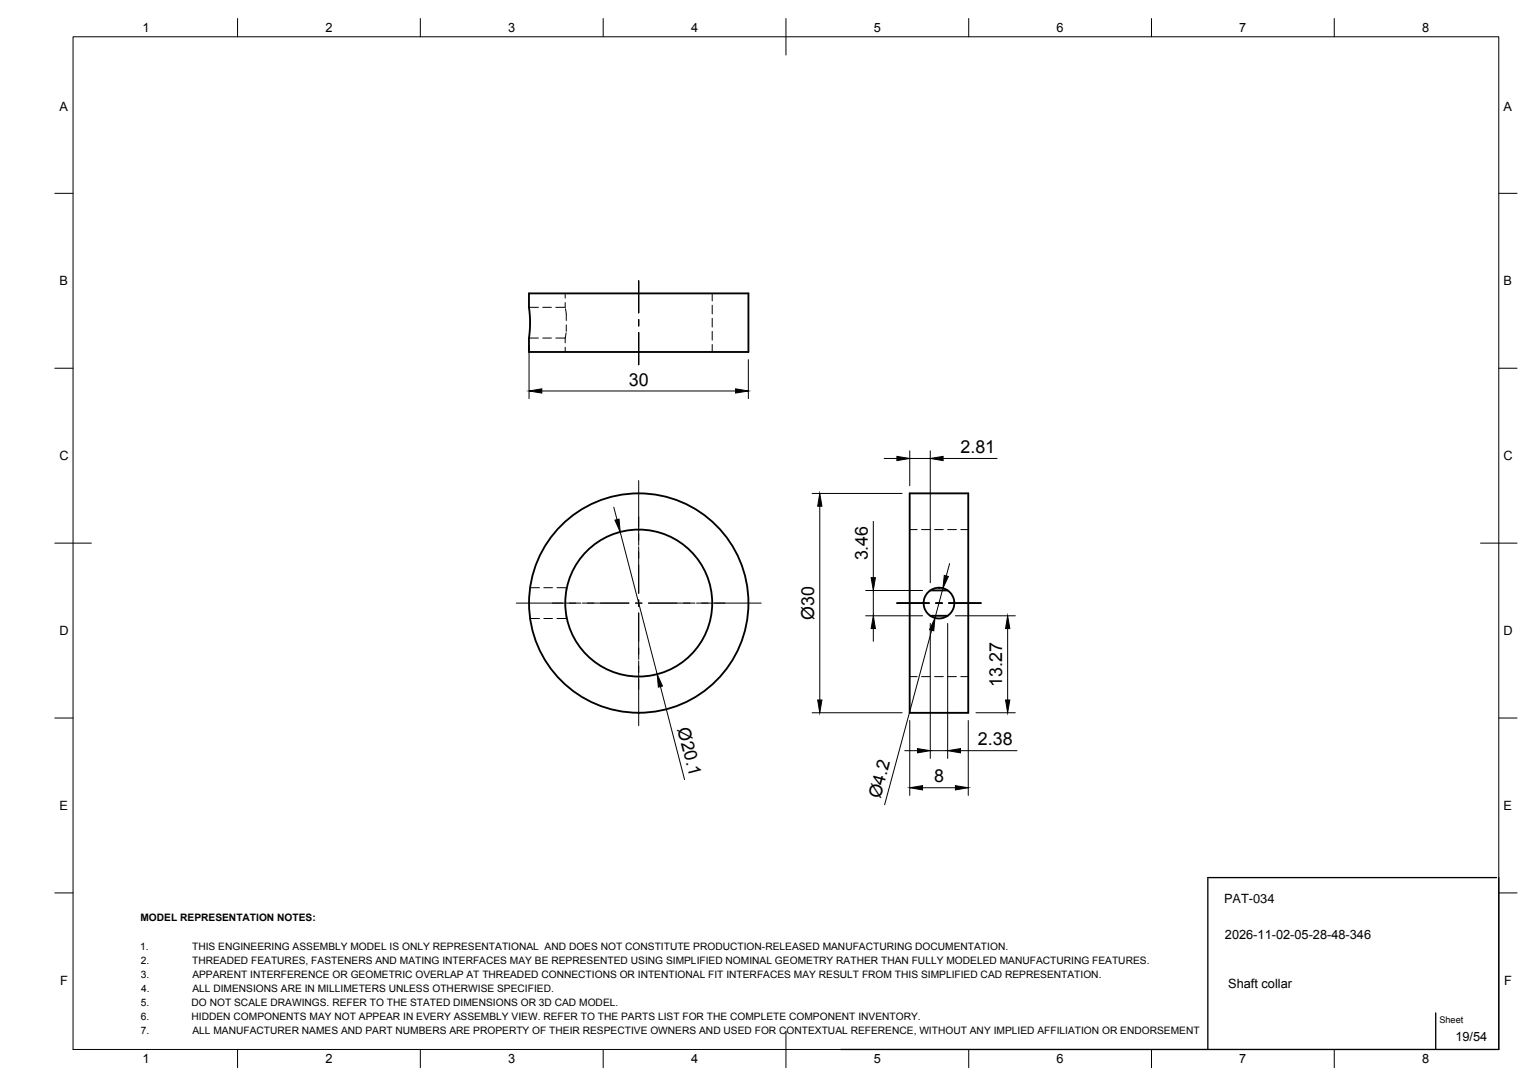
ISO-10303-21;
HEADER;
/* Generated by software containing ST-Developer
 * from STEP Tools, Inc. (www.steptools.com) 
 */

FILE_DESCRIPTION(
/* description */ ('Fatigue rig crank-slider'),
/* implementation_level */ '2;1');

FILE_NAME(
/* name */ 'Shaft collar.step',
/* time_stamp */ '2026-10-28T03:24:50-07:00',
/* author */ (''),
/* organization */ (''),
/* preprocessor_version */ 'ST-DEVELOPER v20.2',
/* originating_system */ 'Autodesk Translation Framework v15.17.0.0',
/* authorisation */ '');

FILE_SCHEMA (('AUTOMOTIVE_DESIGN { 1 0 10303 214 3 1 1 }'));
ENDSEC;

DATA;
#10=MECHANICAL_DESIGN_GEOMETRIC_PRESENTATION_REPRESENTATION('',(#605),#16911);
#439=B_SPLINE_CURVE_WITH_KNOTS('',3,(#14824,#14825,#14826,#14827,#14828,
#14829,#14830,#14831,#14832,#14833,#14834,#14835,#14836,#14837),
 .UNSPECIFIED.,.F.,.F.,(4,2,2,2,2,2,4),(0.756005737987026,0.793568827564645,
0.8729225200542,0.952276212543755,1.03162990503331,1.11098359752287,1.14854668710048),
 .UNSPECIFIED.);
#440=B_SPLINE_CURVE_WITH_KNOTS('',3,(#14843,#14844,#14845,#14846,#14847,
#14848,#14849,#14850,#14851,#14852,#14853,#14854,#14855,#14856,#14857,#14858,
#14859,#14860),.UNSPECIFIED.,.F.,.F.,(4,2,2,2,2,2,2,2,4),(0.,0.0792165807733624,
0.158433161546725,0.23764869707457,0.316864232602414,0.396079768130259,
0.475295303658103,0.554511884431466,0.633728465204828),.UNSPECIFIED.);
#441=B_SPLINE_CURVE_WITH_KNOTS('',3,(#14861,#14862,#14863,#14864,#14865,
#14866,#14867,#14868,#14869,#14870,#14871,#14872,#14873,#14874,#14875,#14876,
#14877,#14878),.UNSPECIFIED.,.F.,.F.,(4,2,2,2,2,2,2,2,4),(0.633728465204828,
0.712945045978191,0.792161626751553,0.871377162279398,0.950592697807242,
1.02980823333509,1.10902376886293,1.18824034963629,1.26745693040966),
 .UNSPECIFIED.);
#442=B_SPLINE_CURVE_WITH_KNOTS('',3,(#14881,#14882,#14883,#14884,#14885,
#14886,#14887,#14888,#14889,#14890,#14891,#14892,#14893,#14894),
 .UNSPECIFIED.,.F.,.F.,(4,2,2,2,2,2,4),(0.121154929624525,0.158718019202141,
0.238071711691697,0.317425404181252,0.396779096670807,0.476132789160362,
0.513695878737981),.UNSPECIFIED.);
#504=SHAPE_REPRESENTATION_RELATIONSHIP('SRR','None',#17145,#554);
#554=ADVANCED_BREP_SHAPE_REPRESENTATION('',(#662),#16874);
#605=STYLED_ITEM('',(#17487),#662);
#662=MANIFOLD_SOLID_BREP('Body1',#8898);
#821=FACE_BOUND('',#2092,.T.);
#822=FACE_BOUND('',#2094,.T.);
#823=FACE_BOUND('',#2096,.T.);
#824=FACE_BOUND('',#2098,.T.);
#1033=PLANE('',#9913);
#1034=PLANE('',#9918);
#1035=PLANE('',#9925);
#1036=PLANE('',#9926);
#1444=FACE_OUTER_BOUND('',#2088,.T.);
#1445=FACE_OUTER_BOUND('',#2089,.T.);
#1446=FACE_OUTER_BOUND('',#2090,.T.);
#1447=FACE_OUTER_BOUND('',#2091,.T.);
#1448=FACE_OUTER_BOUND('',#2093,.T.);
#1449=FACE_OUTER_BOUND('',#2095,.T.);
#1450=FACE_OUTER_BOUND('',#2097,.T.);
#2088=EDGE_LOOP('',(#6950,#6951));
#2089=EDGE_LOOP('',(#6952,#6953,#6954,#6955,#6956,#6957,#6958,#6959,#6960));
#2090=EDGE_LOOP('',(#6961,#6962,#6963));
#2091=EDGE_LOOP('',(#6964,#6965,#6966,#6967));
#2092=EDGE_LOOP('',(#6968,#6969,#6970,#6971));
#2093=EDGE_LOOP('',(#6972,#6973,#6974,#6975));
#2094=EDGE_LOOP('',(#6976,#6977));
#2095=EDGE_LOOP('',(#6978));
#2096=EDGE_LOOP('',(#6979));
#2097=EDGE_LOOP('',(#6980));
#2098=EDGE_LOOP('',(#6981));
#2744=LINE('',#14820,#3390);
#2745=LINE('',#14841,#3391);
#2746=LINE('',#14896,#3392);
#2747=LINE('',#14901,#3393);
#2748=LINE('',#14907,#3394);
#3390=VECTOR('',#11692,1.);
#3391=VECTOR('',#11699,0.21);
#3392=VECTOR('',#11704,1.);
#3393=VECTOR('',#11709,1.005);
#3394=VECTOR('',#11716,1.5);
#3921=CIRCLE('',#9914,0.21);
#3922=CIRCLE('',#9916,0.21);
#3923=CIRCLE('',#9917,0.21);
#3924=CIRCLE('',#9920,1.005);
#3925=CIRCLE('',#9921,1.005);
#3926=CIRCLE('',#9923,1.5);
#3927=CIRCLE('',#9924,1.5);
#4475=VERTEX_POINT('',#14818);
#4476=VERTEX_POINT('',#14819);
#4477=VERTEX_POINT('',#14823);
#4478=VERTEX_POINT('',#14838);
#4479=VERTEX_POINT('',#14840);
#4480=VERTEX_POINT('',#14842);
#4481=VERTEX_POINT('',#14879);
#4482=VERTEX_POINT('',#14898);
#4483=VERTEX_POINT('',#14900);
#4484=VERTEX_POINT('',#14904);
#4485=VERTEX_POINT('',#14906);
#5373=EDGE_CURVE('',#4475,#4476,#2744,.T.);
#5374=EDGE_CURVE('',#4475,#4476,#3921,.T.);
#5375=EDGE_CURVE('',#4477,#4475,#439,.T.);
#5376=EDGE_CURVE('',#4478,#4477,#3922,.T.);
#5377=EDGE_CURVE('',#4478,#4479,#2745,.T.);
#5378=EDGE_CURVE('',#4480,#4479,#440,.T.);
#5379=EDGE_CURVE('',#4479,#4480,#441,.T.);
#5380=EDGE_CURVE('',#4481,#4478,#3923,.T.);
#5381=EDGE_CURVE('',#4476,#4481,#442,.T.);
#5382=EDGE_CURVE('',#4481,#4477,#2746,.T.);
#5383=EDGE_CURVE('',#4482,#4482,#3924,.T.);
#5384=EDGE_CURVE('',#4482,#4483,#2747,.T.);
#5385=EDGE_CURVE('',#4483,#4483,#3925,.T.);
#5386=EDGE_CURVE('',#4484,#4484,#3926,.T.);
#5387=EDGE_CURVE('',#4484,#4485,#2748,.T.);
#5388=EDGE_CURVE('',#4485,#4485,#3927,.T.);
#6950=ORIENTED_EDGE('',*,*,#5373,.F.);
#6951=ORIENTED_EDGE('',*,*,#5374,.T.);
#6952=ORIENTED_EDGE('',*,*,#5375,.F.);
#6953=ORIENTED_EDGE('',*,*,#5376,.F.);
#6954=ORIENTED_EDGE('',*,*,#5377,.T.);
#6955=ORIENTED_EDGE('',*,*,#5378,.F.);
#6956=ORIENTED_EDGE('',*,*,#5379,.F.);
#6957=ORIENTED_EDGE('',*,*,#5377,.F.);
#6958=ORIENTED_EDGE('',*,*,#5380,.F.);
#6959=ORIENTED_EDGE('',*,*,#5381,.F.);
#6960=ORIENTED_EDGE('',*,*,#5374,.F.);
#6961=ORIENTED_EDGE('',*,*,#5382,.F.);
#6962=ORIENTED_EDGE('',*,*,#5380,.T.);
#6963=ORIENTED_EDGE('',*,*,#5376,.T.);
#6964=ORIENTED_EDGE('',*,*,#5383,.F.);
#6965=ORIENTED_EDGE('',*,*,#5384,.T.);
#6966=ORIENTED_EDGE('',*,*,#5385,.T.);
#6967=ORIENTED_EDGE('',*,*,#5384,.F.);
#6968=ORIENTED_EDGE('',*,*,#5381,.T.);
#6969=ORIENTED_EDGE('',*,*,#5382,.T.);
#6970=ORIENTED_EDGE('',*,*,#5375,.T.);
#6971=ORIENTED_EDGE('',*,*,#5373,.T.);
#6972=ORIENTED_EDGE('',*,*,#5386,.F.);
#6973=ORIENTED_EDGE('',*,*,#5387,.T.);
#6974=ORIENTED_EDGE('',*,*,#5388,.T.);
#6975=ORIENTED_EDGE('',*,*,#5387,.F.);
#6976=ORIENTED_EDGE('',*,*,#5378,.T.);
#6977=ORIENTED_EDGE('',*,*,#5379,.T.);
#6978=ORIENTED_EDGE('',*,*,#5386,.T.);
#6979=ORIENTED_EDGE('',*,*,#5383,.T.);
#6980=ORIENTED_EDGE('',*,*,#5388,.F.);
#6981=ORIENTED_EDGE('',*,*,#5385,.F.);
#8278=CYLINDRICAL_SURFACE('',#9915,0.21);
#8279=CYLINDRICAL_SURFACE('',#9919,1.005);
#8280=CYLINDRICAL_SURFACE('',#9922,1.5);
#8582=ADVANCED_FACE('',(#1444),#1033,.T.);
#8583=ADVANCED_FACE('',(#1445),#8278,.F.);
#8584=ADVANCED_FACE('',(#1446),#1034,.T.);
#8585=ADVANCED_FACE('',(#1447,#821),#8279,.F.);
#8586=ADVANCED_FACE('',(#1448,#822),#8280,.T.);
#8587=ADVANCED_FACE('',(#1449,#823),#1035,.T.);
#8588=ADVANCED_FACE('',(#1450,#824),#1036,.F.);
#8898=CLOSED_SHELL('',(#8582,#8583,#8584,#8585,#8586,#8587,#8588));
#9912=AXIS2_PLACEMENT_3D('',#14816,#11688,#11689);
#9913=AXIS2_PLACEMENT_3D('',#14817,#11690,#11691);
#9914=AXIS2_PLACEMENT_3D('',#14821,#11693,#11694);
#9915=AXIS2_PLACEMENT_3D('',#14822,#11695,#11696);
#9916=AXIS2_PLACEMENT_3D('',#14839,#11697,#11698);
#9917=AXIS2_PLACEMENT_3D('',#14880,#11700,#11701);
#9918=AXIS2_PLACEMENT_3D('',#14895,#11702,#11703);
#9919=AXIS2_PLACEMENT_3D('',#14897,#11705,#11706);
#9920=AXIS2_PLACEMENT_3D('',#14899,#11707,#11708);
#9921=AXIS2_PLACEMENT_3D('',#14902,#11710,#11711);
#9922=AXIS2_PLACEMENT_3D('',#14903,#11712,#11713);
#9923=AXIS2_PLACEMENT_3D('',#14905,#11714,#11715);
#9924=AXIS2_PLACEMENT_3D('',#14908,#11717,#11718);
#9925=AXIS2_PLACEMENT_3D('',#14909,#11719,#11720);
#9926=AXIS2_PLACEMENT_3D('',#14910,#11721,#11722);
#11688=DIRECTION('axis',(0.,0.,1.));
#11689=DIRECTION('refdir',(1.,0.,0.));
#11690=DIRECTION('center_axis',(0.,0.,1.));
#11691=DIRECTION('ref_axis',(1.,0.,0.));
#11692=DIRECTION('',(0.,1.,0.));
#11693=DIRECTION('center_axis',(0.,0.,1.));
#11694=DIRECTION('ref_axis',(1.,0.,0.));
#11695=DIRECTION('center_axis',(0.,0.,1.));
#11696=DIRECTION('ref_axis',(1.,0.,0.));
#11697=DIRECTION('center_axis',(0.,0.,1.));
#11698=DIRECTION('ref_axis',(1.,0.,0.));
#11699=DIRECTION('',(0.,0.,1.));
#11700=DIRECTION('center_axis',(0.,0.,1.));
#11701=DIRECTION('ref_axis',(1.,0.,0.));
#11702=DIRECTION('center_axis',(0.,0.,1.));
#11703=DIRECTION('ref_axis',(1.,0.,0.));
#11704=DIRECTION('',(0.,-1.,0.));
#11705=DIRECTION('center_axis',(0.,1.,0.));
#11706=DIRECTION('ref_axis',(1.,0.,0.));
#11707=DIRECTION('center_axis',(0.,-1.,0.));
#11708=DIRECTION('ref_axis',(1.,0.,0.));
#11709=DIRECTION('',(0.,-1.,0.));
#11710=DIRECTION('center_axis',(0.,-1.,0.));
#11711=DIRECTION('ref_axis',(1.,0.,0.));
#11712=DIRECTION('center_axis',(0.,1.,0.));
#11713=DIRECTION('ref_axis',(1.,0.,0.));
#11714=DIRECTION('center_axis',(0.,1.,0.));
#11715=DIRECTION('ref_axis',(1.,0.,0.));
#11716=DIRECTION('',(0.,-1.,0.));
#11717=DIRECTION('center_axis',(0.,1.,0.));
#11718=DIRECTION('ref_axis',(1.,0.,0.));
#11719=DIRECTION('center_axis',(0.,1.,0.));
#11720=DIRECTION('ref_axis',(1.,0.,0.));
#11721=DIRECTION('center_axis',(0.,1.,0.));
#11722=DIRECTION('ref_axis',(1.,0.,0.));
#14816=CARTESIAN_POINT('',(0.,0.,0.));
#14817=CARTESIAN_POINT('Origin',(0.,-17.05,12.99));
#14818=CARTESIAN_POINT('',(0.172988438920051,-17.1690588089979,12.99));
#14819=CARTESIAN_POINT('',(0.172988438920051,-16.9309411910021,12.99));
#14820=CARTESIAN_POINT('',(0.172988438920051,-17.45,12.99));
#14821=CARTESIAN_POINT('Origin',(0.,-17.05,12.99));
#14822=CARTESIAN_POINT('Origin',(0.,-17.05,12.99));
#14823=CARTESIAN_POINT('',(-0.172988438920051,-17.1690588089979,12.99));
#14824=CARTESIAN_POINT('Ctrl Pts',(-0.172988438920049,-17.1690588089979,
12.99));
#14825=CARTESIAN_POINT('Ctrl Pts',(-0.165594865311309,-17.1798014223953,
12.9912919219764));
#14826=CARTESIAN_POINT('Ctrl Pts',(-0.157297138725604,-17.1896877093727,
12.992653949439));
#14827=CARTESIAN_POINT('Ctrl Pts',(-0.129892073845076,-17.2170927742533,
12.9967480843909));
#14828=CARTESIAN_POINT('Ctrl Pts',(-0.106330167759284,-17.233242056333,
12.9996958932764));
#14829=CARTESIAN_POINT('Ctrl Pts',(-0.0546129046324093,-17.2546977939649,
13.0038502947236));
#14830=CARTESIAN_POINT('Ctrl Pts',(-0.0264512308298518,-17.26,13.005));
#14831=CARTESIAN_POINT('Ctrl Pts',(0.0264512308298517,-17.26,13.005));
#14832=CARTESIAN_POINT('Ctrl Pts',(0.0546129046324092,-17.2546977939649,
13.0038502947236));
#14833=CARTESIAN_POINT('Ctrl Pts',(0.106330167759284,-17.233242056333,12.9996958932764));
#14834=CARTESIAN_POINT('Ctrl Pts',(0.129892073845076,-17.2170927742533,
12.9967480843909));
#14835=CARTESIAN_POINT('Ctrl Pts',(0.157297138725604,-17.1896877093727,
12.9926539494391));
#14836=CARTESIAN_POINT('Ctrl Pts',(0.165594865311311,-17.1798014223953,
12.9912919219764));
#14837=CARTESIAN_POINT('Ctrl Pts',(0.17298843892005,-17.1690588089979,12.99));
#14838=CARTESIAN_POINT('',(-0.21,-17.05,12.99));
#14839=CARTESIAN_POINT('Origin',(0.,-17.05,12.99));
#14840=CARTESIAN_POINT('',(-0.21,-17.05,13.4852272553384));
#14841=CARTESIAN_POINT('',(-0.21,-17.05,12.99));
#14842=CARTESIAN_POINT('',(0.21,-17.05,13.4852272553384));
#14843=CARTESIAN_POINT('Ctrl Pts',(0.21,-17.05,13.4852272553384));
#14844=CARTESIAN_POINT('Ctrl Pts',(0.21,-17.0764055269245,13.4852272553384));
#14845=CARTESIAN_POINT('Ctrl Pts',(0.204715737269596,-17.1045470740907,
13.4860041595441));
#14846=CARTESIAN_POINT('Ctrl Pts',(0.183273763036332,-17.1562762689051,
13.4888007328232));
#14847=CARTESIAN_POINT('Ctrl Pts',(0.167117923970393,-17.179866924128,13.4907789715758));
#14848=CARTESIAN_POINT('Ctrl Pts',(0.129867169887369,-17.217117678211,13.4944848114133));
#14849=CARTESIAN_POINT('Ctrl Pts',(0.106276408305765,-17.2332737100014,
13.4964545565713));
#14850=CARTESIAN_POINT('Ctrl Pts',(0.0545468514058993,-17.2547158248262,
13.4992316551565));
#14851=CARTESIAN_POINT('Ctrl Pts',(0.0264051785092816,-17.26,13.5));
#14852=CARTESIAN_POINT('Ctrl Pts',(-0.0264051785092815,-17.26,13.5));
#14853=CARTESIAN_POINT('Ctrl Pts',(-0.0545468514058992,-17.2547158248262,
13.4992316551565));
#14854=CARTESIAN_POINT('Ctrl Pts',(-0.106276408305765,-17.2332737100014,
13.4964545565713));
#14855=CARTESIAN_POINT('Ctrl Pts',(-0.129867169887368,-17.217117678211,
13.4944848114133));
#14856=CARTESIAN_POINT('Ctrl Pts',(-0.167117923970393,-17.179866924128,
13.4907789715758));
#14857=CARTESIAN_POINT('Ctrl Pts',(-0.183273763036332,-17.1562762689051,
13.4888007328232));
#14858=CARTESIAN_POINT('Ctrl Pts',(-0.204715737269596,-17.1045470740907,
13.4860041595441));
#14859=CARTESIAN_POINT('Ctrl Pts',(-0.21,-17.0764055269245,13.4852272553384));
#14860=CARTESIAN_POINT('Ctrl Pts',(-0.21,-17.05,13.4852272553384));
#14861=CARTESIAN_POINT('Ctrl Pts',(-0.21,-17.05,13.4852272553384));
#14862=CARTESIAN_POINT('Ctrl Pts',(-0.21,-17.0235944730756,13.4852272553384));
#14863=CARTESIAN_POINT('Ctrl Pts',(-0.204715737269596,-16.9954529259093,
13.4860041595441));
#14864=CARTESIAN_POINT('Ctrl Pts',(-0.183273763036332,-16.9437237310949,
13.4888007328232));
#14865=CARTESIAN_POINT('Ctrl Pts',(-0.167117923970393,-16.920133075872,
13.4907789715758));
#14866=CARTESIAN_POINT('Ctrl Pts',(-0.129867169887369,-16.882882321789,
13.4944848114133));
#14867=CARTESIAN_POINT('Ctrl Pts',(-0.106276408305765,-16.8667262899986,
13.4964545565713));
#14868=CARTESIAN_POINT('Ctrl Pts',(-0.0545468514058993,-16.8452841751738,
13.4992316551565));
#14869=CARTESIAN_POINT('Ctrl Pts',(-0.0264051785092816,-16.84,13.5));
#14870=CARTESIAN_POINT('Ctrl Pts',(0.0264051785092815,-16.84,13.5));
#14871=CARTESIAN_POINT('Ctrl Pts',(0.0545468514058992,-16.8452841751738,
13.4992316551565));
#14872=CARTESIAN_POINT('Ctrl Pts',(0.106276408305765,-16.8667262899986,
13.4964545565713));
#14873=CARTESIAN_POINT('Ctrl Pts',(0.129867169887368,-16.882882321789,13.4944848114133));
#14874=CARTESIAN_POINT('Ctrl Pts',(0.167117923970393,-16.920133075872,13.4907789715758));
#14875=CARTESIAN_POINT('Ctrl Pts',(0.183273763036332,-16.9437237310949,
13.4888007328232));
#14876=CARTESIAN_POINT('Ctrl Pts',(0.204715737269596,-16.9954529259093,
13.4860041595441));
#14877=CARTESIAN_POINT('Ctrl Pts',(0.21,-17.0235944730756,13.4852272553384));
#14878=CARTESIAN_POINT('Ctrl Pts',(0.21,-17.05,13.4852272553384));
#14879=CARTESIAN_POINT('',(-0.172988438920051,-16.9309411910021,12.99));
#14880=CARTESIAN_POINT('Origin',(0.,-17.05,12.99));
#14881=CARTESIAN_POINT('Ctrl Pts',(0.17298843892005,-16.9309411910021,12.99));
#14882=CARTESIAN_POINT('Ctrl Pts',(0.165594865311311,-16.9201985776047,
12.9912919219764));
#14883=CARTESIAN_POINT('Ctrl Pts',(0.157297138725604,-16.9103122906273,
12.992653949439));
#14884=CARTESIAN_POINT('Ctrl Pts',(0.129892073845076,-16.8829072257467,
12.9967480843909));
#14885=CARTESIAN_POINT('Ctrl Pts',(0.106330167759284,-16.8667579436671,
12.9996958932764));
#14886=CARTESIAN_POINT('Ctrl Pts',(0.0546129046324093,-16.8453022060351,
13.0038502947236));
#14887=CARTESIAN_POINT('Ctrl Pts',(0.0264512308298517,-16.84,13.005));
#14888=CARTESIAN_POINT('Ctrl Pts',(-0.0264512308298517,-16.84,13.005));
#14889=CARTESIAN_POINT('Ctrl Pts',(-0.054612904632409,-16.8453022060351,
13.0038502947236));
#14890=CARTESIAN_POINT('Ctrl Pts',(-0.106330167759284,-16.8667579436671,
12.9996958932764));
#14891=CARTESIAN_POINT('Ctrl Pts',(-0.129892073845076,-16.8829072257467,
12.9967480843909));
#14892=CARTESIAN_POINT('Ctrl Pts',(-0.157297138725604,-16.9103122906273,
12.9926539494391));
#14893=CARTESIAN_POINT('Ctrl Pts',(-0.165594865311311,-16.9201985776047,
12.9912919219764));
#14894=CARTESIAN_POINT('Ctrl Pts',(-0.17298843892005,-16.9309411910021,
12.99));
#14895=CARTESIAN_POINT('Origin',(0.,-17.05,12.99));
#14896=CARTESIAN_POINT('',(-0.172988438920051,-17.45,12.99));
#14897=CARTESIAN_POINT('Origin',(0.,-17.45,12.));
#14898=CARTESIAN_POINT('',(-1.005,-16.65,12.));
#14899=CARTESIAN_POINT('Origin',(0.,-16.65,12.));
#14900=CARTESIAN_POINT('',(-1.005,-17.45,12.));
#14901=CARTESIAN_POINT('',(-1.005,-17.45,12.));
#14902=CARTESIAN_POINT('Origin',(0.,-17.45,12.));
#14903=CARTESIAN_POINT('Origin',(0.,-17.45,12.));
#14904=CARTESIAN_POINT('',(-1.5,-16.65,12.));
#14905=CARTESIAN_POINT('Origin',(0.,-16.65,12.));
#14906=CARTESIAN_POINT('',(-1.5,-17.45,12.));
#14907=CARTESIAN_POINT('',(-1.5,-17.45,12.));
#14908=CARTESIAN_POINT('Origin',(0.,-17.45,12.));
#14909=CARTESIAN_POINT('Origin',(0.,-16.65,12.));
#14910=CARTESIAN_POINT('Origin',(0.,-17.45,12.));
#16815=UNCERTAINTY_MEASURE_WITH_UNIT(LENGTH_MEASURE(0.001),#16912,
'DISTANCE_ACCURACY_VALUE',
'Maximum model space distance between geometric entities at asserted c
onnectivities');
#16852=UNCERTAINTY_MEASURE_WITH_UNIT(LENGTH_MEASURE(0.001),#16912,
'DISTANCE_ACCURACY_VALUE',
'Maximum model space distance between geometric entities at asserted c
onnectivities');
#16874=(
GEOMETRIC_REPRESENTATION_CONTEXT(3)
GLOBAL_UNCERTAINTY_ASSIGNED_CONTEXT((#16815))
GLOBAL_UNIT_ASSIGNED_CONTEXT((#16912,#16914,#16915))
REPRESENTATION_CONTEXT('','3D')
);
#16911=(
GEOMETRIC_REPRESENTATION_CONTEXT(3)
GLOBAL_UNCERTAINTY_ASSIGNED_CONTEXT((#16852))
GLOBAL_UNIT_ASSIGNED_CONTEXT((#16912,#16914,#16915))
REPRESENTATION_CONTEXT('','3D')
);
#16912=(
LENGTH_UNIT()
NAMED_UNIT(*)
SI_UNIT(.CENTI.,.METRE.)
);
#16914=(
NAMED_UNIT(*)
PLANE_ANGLE_UNIT()
SI_UNIT($,.RADIAN.)
);
#16915=(
NAMED_UNIT(*)
SI_UNIT($,.STERADIAN.)
SOLID_ANGLE_UNIT()
);
#16937=SHAPE_DEFINITION_REPRESENTATION(#16997,#17145);
#16997=PRODUCT_DEFINITION_SHAPE('',$,#17204);
#17145=SHAPE_REPRESENTATION('',(#9912),#16874);
#17182=PRODUCT_DEFINITION_CONTEXT('part definition',#17358,'design');
#17204=PRODUCT_DEFINITION('Shaft collar','Shaft collar',#17262,#17182);
#17262=PRODUCT_DEFINITION_FORMATION('',$,#17381);
#17358=APPLICATION_CONTEXT(
'Core Data for Automotive Mechanical Design Process');
#17359=PRODUCT_CONTEXT('part definition',#17358,'mechanical');
#17381=PRODUCT('Shaft collar','Shaft collar','Shaft collar',(#17359));
#17481=COLOUR_RGB('Grey',0.48,0.52,0.57);
#17482=FILL_AREA_STYLE_COLOUR('',#17481);
#17483=FILL_AREA_STYLE('',(#17482));
#17484=SURFACE_STYLE_FILL_AREA(#17483);
#17485=SURFACE_SIDE_STYLE('',(#17484));
#17486=SURFACE_STYLE_USAGE(.BOTH.,#17485);
#17487=PRESENTATION_STYLE_ASSIGNMENT((#17486));
ENDSEC;
END-ISO-10303-21;
